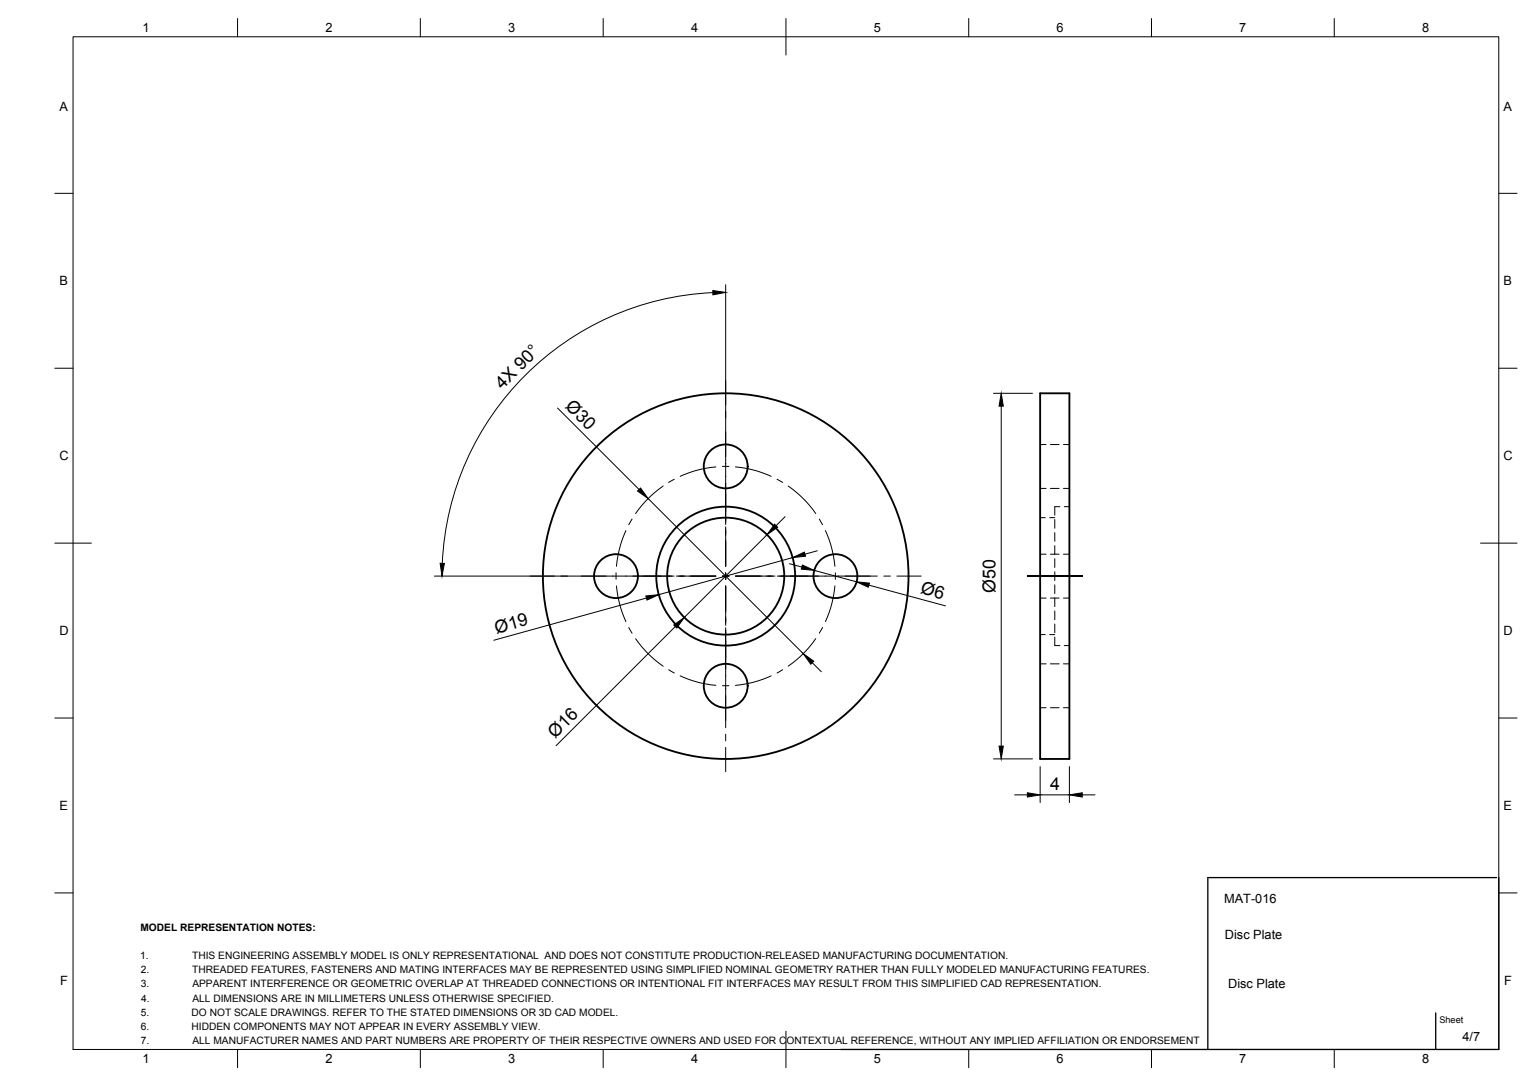
ISO-10303-21;
HEADER;
/* Generated by software containing ST-Developer
 * from STEP Tools, Inc. (www.steptools.com) 
 */

FILE_DESCRIPTION(
/* description */ ('STEP AP214'),
/* implementation_level */ '2;1');

FILE_NAME(
/* name */ 'Disc Plate.step',
/* time_stamp */ '2026-11-14T06:10:26-08:00',
/* author */ (''),
/* organization */ (''),
/* preprocessor_version */ 'ST-DEVELOPER v20.2',
/* originating_system */ 'Autodesk Translation Framework v15.17.0.0',
/* authorisation */ '');

FILE_SCHEMA (('AUTOMOTIVE_DESIGN { 1 0 10303 214 3 1 1 }'));
ENDSEC;

DATA;
#10=MECHANICAL_DESIGN_GEOMETRIC_PRESENTATION_REPRESENTATION('',(#168),#10413);
#152=SHAPE_REPRESENTATION_RELATIONSHIP('SRR','None',#10457,#160);
#160=ADVANCED_BREP_SHAPE_REPRESENTATION('',(#176),#10409);
#168=STYLED_ITEM('',(#10504),#176);
#176=MANIFOLD_SOLID_BREP('Body1',#5303);
#203=FACE_BOUND('',#838,.T.);
#204=FACE_BOUND('',#839,.T.);
#205=FACE_BOUND('',#840,.T.);
#206=FACE_BOUND('',#841,.T.);
#207=FACE_BOUND('',#842,.T.);
#208=FACE_BOUND('',#844,.T.);
#209=FACE_BOUND('',#845,.T.);
#210=FACE_BOUND('',#846,.T.);
#211=FACE_BOUND('',#847,.T.);
#212=FACE_BOUND('',#848,.T.);
#213=FACE_BOUND('',#850,.T.);
#253=PLANE('',#6073);
#254=PLANE('',#6074);
#255=PLANE('',#6075);
#517=FACE_OUTER_BOUND('',#830,.T.);
#518=FACE_OUTER_BOUND('',#831,.T.);
#519=FACE_OUTER_BOUND('',#832,.T.);
#520=FACE_OUTER_BOUND('',#833,.T.);
#521=FACE_OUTER_BOUND('',#834,.T.);
#522=FACE_OUTER_BOUND('',#835,.T.);
#523=FACE_OUTER_BOUND('',#836,.T.);
#524=FACE_OUTER_BOUND('',#837,.T.);
#525=FACE_OUTER_BOUND('',#843,.T.);
#526=FACE_OUTER_BOUND('',#849,.T.);
#830=EDGE_LOOP('',(#4568,#4569,#4570,#4571));
#831=EDGE_LOOP('',(#4572,#4573,#4574,#4575));
#832=EDGE_LOOP('',(#4576,#4577,#4578,#4579));
#833=EDGE_LOOP('',(#4580,#4581,#4582,#4583));
#834=EDGE_LOOP('',(#4584,#4585,#4586,#4587));
#835=EDGE_LOOP('',(#4588,#4589,#4590,#4591));
#836=EDGE_LOOP('',(#4592,#4593,#4594,#4595));
#837=EDGE_LOOP('',(#4596));
#838=EDGE_LOOP('',(#4597));
#839=EDGE_LOOP('',(#4598));
#840=EDGE_LOOP('',(#4599));
#841=EDGE_LOOP('',(#4600));
#842=EDGE_LOOP('',(#4601));
#843=EDGE_LOOP('',(#4602));
#844=EDGE_LOOP('',(#4603));
#845=EDGE_LOOP('',(#4604));
#846=EDGE_LOOP('',(#4605));
#847=EDGE_LOOP('',(#4606));
#848=EDGE_LOOP('',(#4607));
#849=EDGE_LOOP('',(#4608));
#850=EDGE_LOOP('',(#4609));
#1135=LINE('',#9366,#1426);
#1136=LINE('',#9372,#1427);
#1137=LINE('',#9378,#1428);
#1138=LINE('',#9384,#1429);
#1139=LINE('',#9390,#1430);
#1140=LINE('',#9396,#1431);
#1141=LINE('',#9402,#1432);
#1426=VECTOR('',#7707,8.);
#1427=VECTOR('',#7714,25.);
#1428=VECTOR('',#7721,3.);
#1429=VECTOR('',#7728,3.);
#1430=VECTOR('',#7735,3.);
#1431=VECTOR('',#7742,3.);
#1432=VECTOR('',#7749,9.5);
#1884=CIRCLE('',#6053,8.);
#1885=CIRCLE('',#6054,8.);
#1886=CIRCLE('',#6056,25.);
#1887=CIRCLE('',#6057,25.);
#1888=CIRCLE('',#6059,3.);
#1889=CIRCLE('',#6060,3.);
#1890=CIRCLE('',#6062,3.);
#1891=CIRCLE('',#6063,3.);
#1892=CIRCLE('',#6065,3.);
#1893=CIRCLE('',#6066,3.);
#1894=CIRCLE('',#6068,3.);
#1895=CIRCLE('',#6069,3.);
#1896=CIRCLE('',#6071,9.5);
#1897=CIRCLE('',#6072,9.5);
#2361=VERTEX_POINT('',#9363);
#2362=VERTEX_POINT('',#9365);
#2363=VERTEX_POINT('',#9369);
#2364=VERTEX_POINT('',#9371);
#2365=VERTEX_POINT('',#9375);
#2366=VERTEX_POINT('',#9377);
#2367=VERTEX_POINT('',#9381);
#2368=VERTEX_POINT('',#9383);
#2369=VERTEX_POINT('',#9387);
#2370=VERTEX_POINT('',#9389);
#2371=VERTEX_POINT('',#9393);
#2372=VERTEX_POINT('',#9395);
#2373=VERTEX_POINT('',#9399);
#2374=VERTEX_POINT('',#9401);
#3109=EDGE_CURVE('',#2361,#2361,#1884,.T.);
#3110=EDGE_CURVE('',#2361,#2362,#1135,.T.);
#3111=EDGE_CURVE('',#2362,#2362,#1885,.T.);
#3112=EDGE_CURVE('',#2363,#2363,#1886,.T.);
#3113=EDGE_CURVE('',#2363,#2364,#1136,.T.);
#3114=EDGE_CURVE('',#2364,#2364,#1887,.T.);
#3115=EDGE_CURVE('',#2365,#2365,#1888,.T.);
#3116=EDGE_CURVE('',#2365,#2366,#1137,.T.);
#3117=EDGE_CURVE('',#2366,#2366,#1889,.T.);
#3118=EDGE_CURVE('',#2367,#2367,#1890,.T.);
#3119=EDGE_CURVE('',#2367,#2368,#1138,.T.);
#3120=EDGE_CURVE('',#2368,#2368,#1891,.T.);
#3121=EDGE_CURVE('',#2369,#2369,#1892,.T.);
#3122=EDGE_CURVE('',#2369,#2370,#1139,.T.);
#3123=EDGE_CURVE('',#2370,#2370,#1893,.T.);
#3124=EDGE_CURVE('',#2371,#2371,#1894,.T.);
#3125=EDGE_CURVE('',#2371,#2372,#1140,.T.);
#3126=EDGE_CURVE('',#2372,#2372,#1895,.T.);
#3127=EDGE_CURVE('',#2373,#2373,#1896,.T.);
#3128=EDGE_CURVE('',#2373,#2374,#1141,.T.);
#3129=EDGE_CURVE('',#2374,#2374,#1897,.T.);
#4568=ORIENTED_EDGE('',*,*,#3109,.T.);
#4569=ORIENTED_EDGE('',*,*,#3110,.T.);
#4570=ORIENTED_EDGE('',*,*,#3111,.F.);
#4571=ORIENTED_EDGE('',*,*,#3110,.F.);
#4572=ORIENTED_EDGE('',*,*,#3112,.T.);
#4573=ORIENTED_EDGE('',*,*,#3113,.T.);
#4574=ORIENTED_EDGE('',*,*,#3114,.F.);
#4575=ORIENTED_EDGE('',*,*,#3113,.F.);
#4576=ORIENTED_EDGE('',*,*,#3115,.T.);
#4577=ORIENTED_EDGE('',*,*,#3116,.T.);
#4578=ORIENTED_EDGE('',*,*,#3117,.F.);
#4579=ORIENTED_EDGE('',*,*,#3116,.F.);
#4580=ORIENTED_EDGE('',*,*,#3118,.T.);
#4581=ORIENTED_EDGE('',*,*,#3119,.T.);
#4582=ORIENTED_EDGE('',*,*,#3120,.F.);
#4583=ORIENTED_EDGE('',*,*,#3119,.F.);
#4584=ORIENTED_EDGE('',*,*,#3121,.T.);
#4585=ORIENTED_EDGE('',*,*,#3122,.T.);
#4586=ORIENTED_EDGE('',*,*,#3123,.F.);
#4587=ORIENTED_EDGE('',*,*,#3122,.F.);
#4588=ORIENTED_EDGE('',*,*,#3124,.T.);
#4589=ORIENTED_EDGE('',*,*,#3125,.T.);
#4590=ORIENTED_EDGE('',*,*,#3126,.F.);
#4591=ORIENTED_EDGE('',*,*,#3125,.F.);
#4592=ORIENTED_EDGE('',*,*,#3127,.T.);
#4593=ORIENTED_EDGE('',*,*,#3128,.T.);
#4594=ORIENTED_EDGE('',*,*,#3129,.F.);
#4595=ORIENTED_EDGE('',*,*,#3128,.F.);
#4596=ORIENTED_EDGE('',*,*,#3114,.T.);
#4597=ORIENTED_EDGE('',*,*,#3115,.F.);
#4598=ORIENTED_EDGE('',*,*,#3118,.F.);
#4599=ORIENTED_EDGE('',*,*,#3121,.F.);
#4600=ORIENTED_EDGE('',*,*,#3124,.F.);
#4601=ORIENTED_EDGE('',*,*,#3127,.F.);
#4602=ORIENTED_EDGE('',*,*,#3112,.F.);
#4603=ORIENTED_EDGE('',*,*,#3111,.T.);
#4604=ORIENTED_EDGE('',*,*,#3117,.T.);
#4605=ORIENTED_EDGE('',*,*,#3120,.T.);
#4606=ORIENTED_EDGE('',*,*,#3123,.T.);
#4607=ORIENTED_EDGE('',*,*,#3126,.T.);
#4608=ORIENTED_EDGE('',*,*,#3129,.T.);
#4609=ORIENTED_EDGE('',*,*,#3109,.F.);
#4990=CYLINDRICAL_SURFACE('',#6052,8.);
#4991=CYLINDRICAL_SURFACE('',#6055,25.);
#4992=CYLINDRICAL_SURFACE('',#6058,3.);
#4993=CYLINDRICAL_SURFACE('',#6061,3.);
#4994=CYLINDRICAL_SURFACE('',#6064,3.);
#4995=CYLINDRICAL_SURFACE('',#6067,3.);
#4996=CYLINDRICAL_SURFACE('',#6070,9.5);
#5251=ADVANCED_FACE('',(#517),#4990,.F.);
#5252=ADVANCED_FACE('',(#518),#4991,.T.);
#5253=ADVANCED_FACE('',(#519),#4992,.F.);
#5254=ADVANCED_FACE('',(#520),#4993,.F.);
#5255=ADVANCED_FACE('',(#521),#4994,.F.);
#5256=ADVANCED_FACE('',(#522),#4995,.F.);
#5257=ADVANCED_FACE('',(#523),#4996,.F.);
#5258=ADVANCED_FACE('',(#524,#203,#204,#205,#206,#207),#253,.T.);
#5259=ADVANCED_FACE('',(#525,#208,#209,#210,#211,#212),#254,.F.);
#5260=ADVANCED_FACE('',(#526,#213),#255,.T.);
#5303=CLOSED_SHELL('',(#5251,#5252,#5253,#5254,#5255,#5256,#5257,#5258,
#5259,#5260));
#6051=AXIS2_PLACEMENT_3D('',#9361,#7701,#7702);
#6052=AXIS2_PLACEMENT_3D('',#9362,#7703,#7704);
#6053=AXIS2_PLACEMENT_3D('',#9364,#7705,#7706);
#6054=AXIS2_PLACEMENT_3D('',#9367,#7708,#7709);
#6055=AXIS2_PLACEMENT_3D('',#9368,#7710,#7711);
#6056=AXIS2_PLACEMENT_3D('',#9370,#7712,#7713);
#6057=AXIS2_PLACEMENT_3D('',#9373,#7715,#7716);
#6058=AXIS2_PLACEMENT_3D('',#9374,#7717,#7718);
#6059=AXIS2_PLACEMENT_3D('',#9376,#7719,#7720);
#6060=AXIS2_PLACEMENT_3D('',#9379,#7722,#7723);
#6061=AXIS2_PLACEMENT_3D('',#9380,#7724,#7725);
#6062=AXIS2_PLACEMENT_3D('',#9382,#7726,#7727);
#6063=AXIS2_PLACEMENT_3D('',#9385,#7729,#7730);
#6064=AXIS2_PLACEMENT_3D('',#9386,#7731,#7732);
#6065=AXIS2_PLACEMENT_3D('',#9388,#7733,#7734);
#6066=AXIS2_PLACEMENT_3D('',#9391,#7736,#7737);
#6067=AXIS2_PLACEMENT_3D('',#9392,#7738,#7739);
#6068=AXIS2_PLACEMENT_3D('',#9394,#7740,#7741);
#6069=AXIS2_PLACEMENT_3D('',#9397,#7743,#7744);
#6070=AXIS2_PLACEMENT_3D('',#9398,#7745,#7746);
#6071=AXIS2_PLACEMENT_3D('',#9400,#7747,#7748);
#6072=AXIS2_PLACEMENT_3D('',#9403,#7750,#7751);
#6073=AXIS2_PLACEMENT_3D('',#9404,#7752,#7753);
#6074=AXIS2_PLACEMENT_3D('',#9405,#7754,#7755);
#6075=AXIS2_PLACEMENT_3D('',#9406,#7756,#7757);
#7701=DIRECTION('axis',(0.,0.,1.));
#7702=DIRECTION('refdir',(1.,0.,0.));
#7703=DIRECTION('center_axis',(0.,0.,-1.));
#7704=DIRECTION('ref_axis',(-1.,0.,0.));
#7705=DIRECTION('center_axis',(0.,0.,1.));
#7706=DIRECTION('ref_axis',(1.,0.,0.));
#7707=DIRECTION('',(0.,0.,-1.));
#7708=DIRECTION('center_axis',(0.,0.,1.));
#7709=DIRECTION('ref_axis',(1.,0.,0.));
#7710=DIRECTION('center_axis',(0.,0.,-1.));
#7711=DIRECTION('ref_axis',(-1.,0.,0.));
#7712=DIRECTION('center_axis',(0.,0.,1.));
#7713=DIRECTION('ref_axis',(1.,0.,0.));
#7714=DIRECTION('',(0.,0.,1.));
#7715=DIRECTION('center_axis',(0.,0.,1.));
#7716=DIRECTION('ref_axis',(1.,0.,0.));
#7717=DIRECTION('center_axis',(0.,0.,-1.));
#7718=DIRECTION('ref_axis',(-1.,0.,0.));
#7719=DIRECTION('center_axis',(0.,0.,1.));
#7720=DIRECTION('ref_axis',(1.,0.,0.));
#7721=DIRECTION('',(0.,0.,-1.));
#7722=DIRECTION('center_axis',(0.,0.,1.));
#7723=DIRECTION('ref_axis',(1.,0.,0.));
#7724=DIRECTION('center_axis',(0.,0.,-1.));
#7725=DIRECTION('ref_axis',(-1.,0.,0.));
#7726=DIRECTION('center_axis',(0.,0.,1.));
#7727=DIRECTION('ref_axis',(1.,0.,0.));
#7728=DIRECTION('',(0.,0.,-1.));
#7729=DIRECTION('center_axis',(0.,0.,1.));
#7730=DIRECTION('ref_axis',(1.,0.,0.));
#7731=DIRECTION('center_axis',(0.,0.,-1.));
#7732=DIRECTION('ref_axis',(-1.,0.,0.));
#7733=DIRECTION('center_axis',(0.,0.,1.));
#7734=DIRECTION('ref_axis',(1.,0.,0.));
#7735=DIRECTION('',(0.,0.,-1.));
#7736=DIRECTION('center_axis',(0.,0.,1.));
#7737=DIRECTION('ref_axis',(1.,0.,0.));
#7738=DIRECTION('center_axis',(0.,0.,-1.));
#7739=DIRECTION('ref_axis',(-1.,0.,0.));
#7740=DIRECTION('center_axis',(0.,0.,1.));
#7741=DIRECTION('ref_axis',(1.,0.,0.));
#7742=DIRECTION('',(0.,0.,-1.));
#7743=DIRECTION('center_axis',(0.,0.,1.));
#7744=DIRECTION('ref_axis',(1.,0.,0.));
#7745=DIRECTION('center_axis',(0.,0.,-1.));
#7746=DIRECTION('ref_axis',(-1.,0.,0.));
#7747=DIRECTION('center_axis',(0.,0.,1.));
#7748=DIRECTION('ref_axis',(1.,0.,0.));
#7749=DIRECTION('',(0.,0.,-1.));
#7750=DIRECTION('center_axis',(0.,0.,1.));
#7751=DIRECTION('ref_axis',(1.,0.,0.));
#7752=DIRECTION('center_axis',(0.,0.,1.));
#7753=DIRECTION('ref_axis',(1.,0.,0.));
#7754=DIRECTION('center_axis',(0.,0.,1.));
#7755=DIRECTION('ref_axis',(1.,0.,0.));
#7756=DIRECTION('center_axis',(0.,0.,1.));
#7757=DIRECTION('ref_axis',(1.,0.,0.));
#9361=CARTESIAN_POINT('',(0.,0.,0.));
#9362=CARTESIAN_POINT('Origin',(0.,0.,2.));
#9363=CARTESIAN_POINT('',(8.,-9.79717439317883E-16,2.));
#9364=CARTESIAN_POINT('Origin',(0.,0.,2.));
#9365=CARTESIAN_POINT('',(8.,-9.79717439317883E-16,0.));
#9366=CARTESIAN_POINT('',(8.,-9.79717439317883E-16,2.));
#9367=CARTESIAN_POINT('Origin',(0.,0.,0.));
#9368=CARTESIAN_POINT('Origin',(0.,0.,4.));
#9369=CARTESIAN_POINT('',(25.,-3.06161699786838E-15,0.));
#9370=CARTESIAN_POINT('Origin',(0.,0.,0.));
#9371=CARTESIAN_POINT('',(25.,-3.06161699786838E-15,4.));
#9372=CARTESIAN_POINT('',(25.,-3.06161699786838E-15,4.));
#9373=CARTESIAN_POINT('Origin',(0.,0.,4.));
#9374=CARTESIAN_POINT('Origin',(-15.,1.57116660247941E-13,4.));
#9375=CARTESIAN_POINT('',(-12.,1.56749266208197E-13,4.));
#9376=CARTESIAN_POINT('Origin',(-15.,1.57116660247941E-13,4.));
#9377=CARTESIAN_POINT('',(-12.,1.56749266208197E-13,0.));
#9378=CARTESIAN_POINT('',(-12.,1.56749266208197E-13,4.));
#9379=CARTESIAN_POINT('Origin',(-15.,1.57116660247941E-13,0.));
#9380=CARTESIAN_POINT('Origin',(-1.04744440165294E-13,-15.,4.));
#9381=CARTESIAN_POINT('',(2.9999999999999,-15.,4.));
#9382=CARTESIAN_POINT('Origin',(-1.04744440165294E-13,-15.,4.));
#9383=CARTESIAN_POINT('',(2.9999999999999,-15.,0.));
#9384=CARTESIAN_POINT('',(2.9999999999999,-15.,4.));
#9385=CARTESIAN_POINT('Origin',(-1.04744440165294E-13,-15.,0.));
#9386=CARTESIAN_POINT('Origin',(15.,-5.2372220082647E-14,4.));
#9387=CARTESIAN_POINT('',(18.,-5.27396141223912E-14,4.));
#9388=CARTESIAN_POINT('Origin',(15.,-5.2372220082647E-14,4.));
#9389=CARTESIAN_POINT('',(18.,-5.27396141223912E-14,0.));
#9390=CARTESIAN_POINT('',(18.,-5.27396141223912E-14,4.));
#9391=CARTESIAN_POINT('Origin',(15.,-5.2372220082647E-14,0.));
#9392=CARTESIAN_POINT('Origin',(0.,15.,4.));
#9393=CARTESIAN_POINT('',(3.,15.,4.));
#9394=CARTESIAN_POINT('Origin',(0.,15.,4.));
#9395=CARTESIAN_POINT('',(3.,15.,0.));
#9396=CARTESIAN_POINT('',(3.,15.,4.));
#9397=CARTESIAN_POINT('Origin',(0.,15.,0.));
#9398=CARTESIAN_POINT('Origin',(0.,0.,4.));
#9399=CARTESIAN_POINT('',(9.5,-1.16341445918999E-15,4.));
#9400=CARTESIAN_POINT('Origin',(0.,0.,4.));
#9401=CARTESIAN_POINT('',(9.5,-1.16341445918999E-15,2.));
#9402=CARTESIAN_POINT('',(9.5,-1.16341445918999E-15,4.));
#9403=CARTESIAN_POINT('Origin',(0.,0.,2.));
#9404=CARTESIAN_POINT('Origin',(0.,0.,4.));
#9405=CARTESIAN_POINT('Origin',(0.,0.,0.));
#9406=CARTESIAN_POINT('Origin',(0.,0.,2.));
#10399=UNCERTAINTY_MEASURE_WITH_UNIT(LENGTH_MEASURE(0.01),#10414,
'DISTANCE_ACCURACY_VALUE',
'Maximum model space distance between geometric entities at asserted c
onnectivities');
#10403=UNCERTAINTY_MEASURE_WITH_UNIT(LENGTH_MEASURE(0.01),#10414,
'DISTANCE_ACCURACY_VALUE',
'Maximum model space distance between geometric entities at asserted c
onnectivities');
#10409=(
GEOMETRIC_REPRESENTATION_CONTEXT(3)
GLOBAL_UNCERTAINTY_ASSIGNED_CONTEXT((#10399))
GLOBAL_UNIT_ASSIGNED_CONTEXT((#10414,#10416,#10417))
REPRESENTATION_CONTEXT('','3D')
);
#10413=(
GEOMETRIC_REPRESENTATION_CONTEXT(3)
GLOBAL_UNCERTAINTY_ASSIGNED_CONTEXT((#10403))
GLOBAL_UNIT_ASSIGNED_CONTEXT((#10414,#10416,#10417))
REPRESENTATION_CONTEXT('','3D')
);
#10414=(
LENGTH_UNIT()
NAMED_UNIT(*)
SI_UNIT(.MILLI.,.METRE.)
);
#10416=(
NAMED_UNIT(*)
PLANE_ANGLE_UNIT()
SI_UNIT($,.RADIAN.)
);
#10417=(
NAMED_UNIT(*)
SI_UNIT($,.STERADIAN.)
SOLID_ANGLE_UNIT()
);
#10423=SHAPE_DEFINITION_REPRESENTATION(#10432,#10457);
#10432=PRODUCT_DEFINITION_SHAPE('',$,#10467);
#10457=SHAPE_REPRESENTATION('',(#6051),#10409);
#10461=PRODUCT_DEFINITION_CONTEXT('part definition',#10490,'design');
#10467=PRODUCT_DEFINITION('Disc Plate','Disc Plate',#10476,#10461);
#10476=PRODUCT_DEFINITION_FORMATION('',$,#10497);
#10490=APPLICATION_CONTEXT(
'Core Data for Automotive Mechanical Design Process');
#10491=PRODUCT_CONTEXT('part definition',#10490,'mechanical');
#10497=PRODUCT('Disc Plate','Disc Plate',$,(#10491));
#10504=PRESENTATION_STYLE_ASSIGNMENT((#10508));
#10508=SURFACE_STYLE_USAGE(.BOTH.,#10512);
#10512=SURFACE_SIDE_STYLE('',(#10516));
#10516=SURFACE_STYLE_FILL_AREA(#10520);
#10520=FILL_AREA_STYLE('Opaque(227,224,212)',(#10524));
#10524=FILL_AREA_STYLE_COLOUR('Opaque(227,224,212)',#10528);
#10528=COLOUR_RGB('Opaque(227,224,212)',0.890196078431372,0.87843137254902,
0.831372549019608);
ENDSEC;
END-ISO-10303-21;
